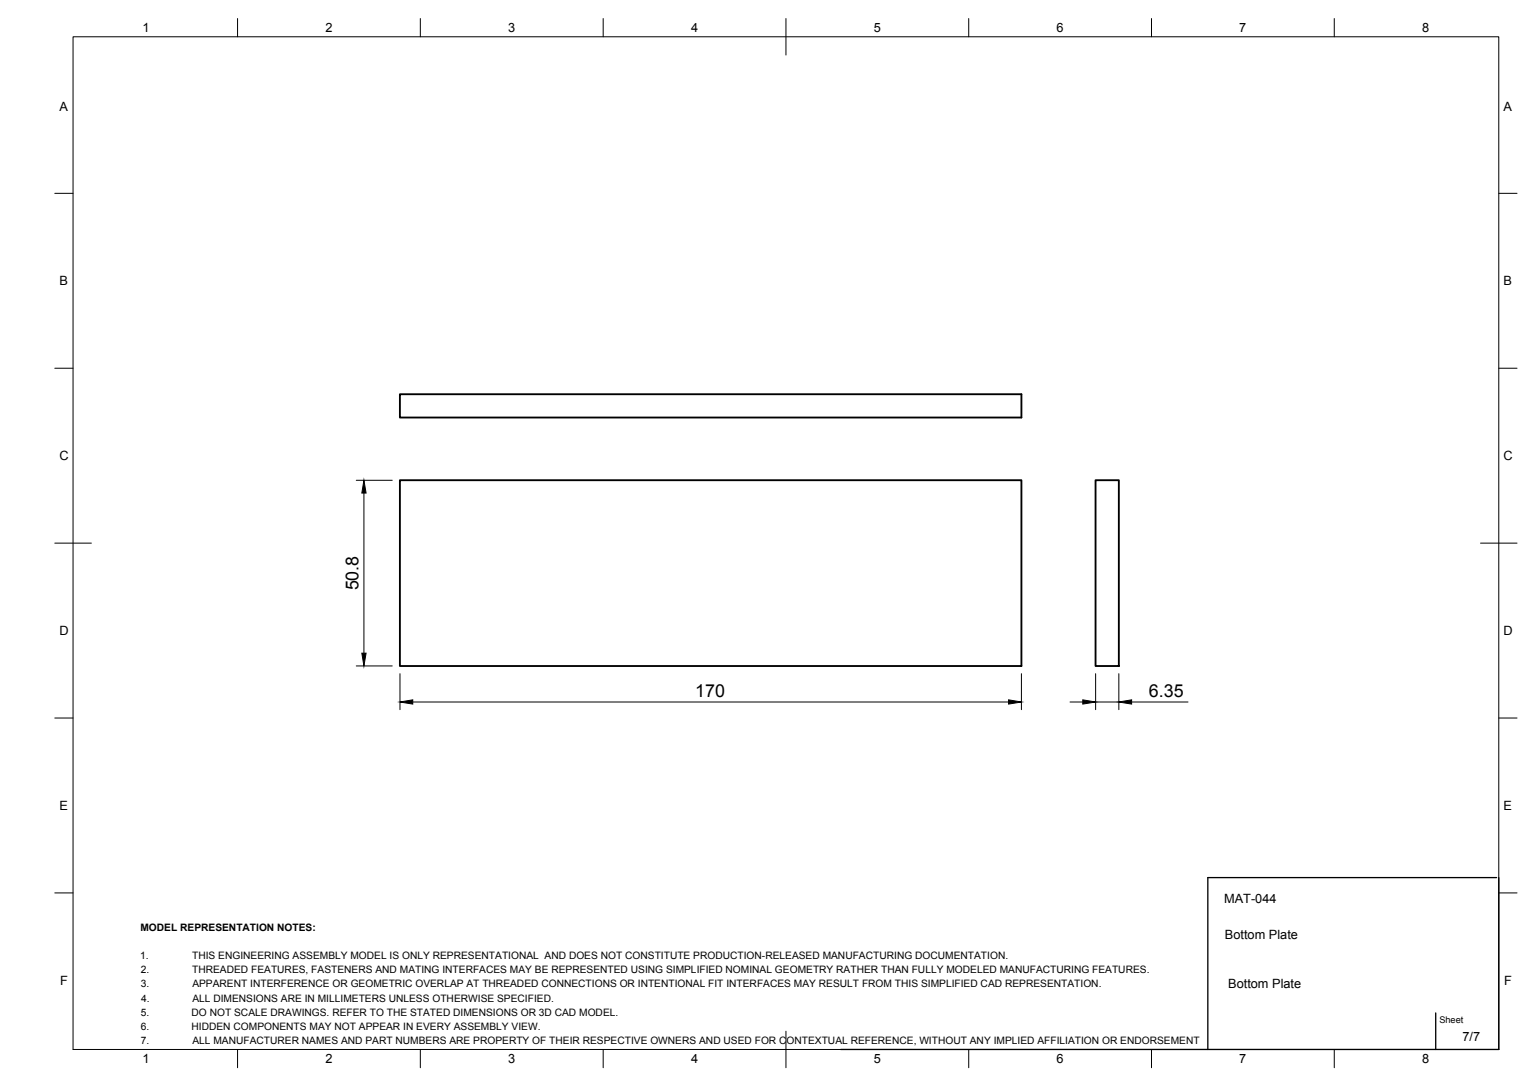
ISO-10303-21;
HEADER;
/* Generated by software containing ST-Developer
 * from STEP Tools, Inc. (www.steptools.com) 
 */

FILE_DESCRIPTION(
/* description */ ('STEP AP214'),
/* implementation_level */ '2;1');

FILE_NAME(
/* name */ 'Bottom Plate.step',
/* time_stamp */ '2026-11-14T22:20:24-08:00',
/* author */ (''),
/* organization */ (''),
/* preprocessor_version */ 'ST-DEVELOPER v20.2',
/* originating_system */ 'Autodesk Translation Framework v15.17.0.0',
/* authorisation */ '');

FILE_SCHEMA (('AUTOMOTIVE_DESIGN { 1 0 10303 214 3 1 1 }'));
ENDSEC;

DATA;
#10=MECHANICAL_DESIGN_GEOMETRIC_PRESENTATION_REPRESENTATION('',(#85),#2794);
#75=SHAPE_REPRESENTATION_RELATIONSHIP('SRR','None',#2830,#80);
#80=ADVANCED_BREP_SHAPE_REPRESENTATION('',(#90),#2792);
#85=STYLED_ITEM('',(#2863),#90);
#90=MANIFOLD_SOLID_BREP('Body1',#1644);
#178=PLANE('',#1823);
#179=PLANE('',#1824);
#180=PLANE('',#1825);
#181=PLANE('',#1826);
#182=PLANE('',#1827);
#183=PLANE('',#1828);
#266=FACE_OUTER_BOUND('',#379,.T.);
#267=FACE_OUTER_BOUND('',#380,.T.);
#268=FACE_OUTER_BOUND('',#381,.T.);
#269=FACE_OUTER_BOUND('',#382,.T.);
#270=FACE_OUTER_BOUND('',#383,.T.);
#271=FACE_OUTER_BOUND('',#384,.T.);
#379=EDGE_LOOP('',(#1490,#1491,#1492,#1493));
#380=EDGE_LOOP('',(#1494,#1495,#1496,#1497));
#381=EDGE_LOOP('',(#1498,#1499,#1500,#1501));
#382=EDGE_LOOP('',(#1502,#1503,#1504,#1505));
#383=EDGE_LOOP('',(#1506,#1507,#1508,#1509));
#384=EDGE_LOOP('',(#1510,#1511,#1512,#1513));
#546=LINE('',#2724,#715);
#547=LINE('',#2726,#716);
#548=LINE('',#2728,#717);
#549=LINE('',#2729,#718);
#550=LINE('',#2732,#719);
#551=LINE('',#2734,#720);
#552=LINE('',#2735,#721);
#553=LINE('',#2738,#722);
#554=LINE('',#2740,#723);
#555=LINE('',#2741,#724);
#556=LINE('',#2743,#725);
#557=LINE('',#2744,#726);
#715=VECTOR('',#2253,1000.);
#716=VECTOR('',#2254,1000.);
#717=VECTOR('',#2255,1000.);
#718=VECTOR('',#2256,1000.);
#719=VECTOR('',#2259,1000.);
#720=VECTOR('',#2260,1000.);
#721=VECTOR('',#2261,1000.);
#722=VECTOR('',#2264,1000.);
#723=VECTOR('',#2265,1000.);
#724=VECTOR('',#2266,1000.);
#725=VECTOR('',#2269,1000.);
#726=VECTOR('',#2270,1000.);
#887=VERTEX_POINT('',#2722);
#888=VERTEX_POINT('',#2723);
#889=VERTEX_POINT('',#2725);
#890=VERTEX_POINT('',#2727);
#891=VERTEX_POINT('',#2731);
#892=VERTEX_POINT('',#2733);
#893=VERTEX_POINT('',#2737);
#894=VERTEX_POINT('',#2739);
#1090=EDGE_CURVE('',#887,#888,#546,.T.);
#1091=EDGE_CURVE('',#889,#888,#547,.T.);
#1092=EDGE_CURVE('',#890,#889,#548,.T.);
#1093=EDGE_CURVE('',#890,#887,#549,.T.);
#1094=EDGE_CURVE('',#888,#891,#550,.T.);
#1095=EDGE_CURVE('',#892,#891,#551,.T.);
#1096=EDGE_CURVE('',#889,#892,#552,.T.);
#1097=EDGE_CURVE('',#891,#893,#553,.T.);
#1098=EDGE_CURVE('',#894,#893,#554,.T.);
#1099=EDGE_CURVE('',#892,#894,#555,.T.);
#1100=EDGE_CURVE('',#893,#887,#556,.T.);
#1101=EDGE_CURVE('',#894,#890,#557,.T.);
#1490=ORIENTED_EDGE('',*,*,#1090,.T.);
#1491=ORIENTED_EDGE('',*,*,#1091,.F.);
#1492=ORIENTED_EDGE('',*,*,#1092,.F.);
#1493=ORIENTED_EDGE('',*,*,#1093,.T.);
#1494=ORIENTED_EDGE('',*,*,#1094,.T.);
#1495=ORIENTED_EDGE('',*,*,#1095,.F.);
#1496=ORIENTED_EDGE('',*,*,#1096,.F.);
#1497=ORIENTED_EDGE('',*,*,#1091,.T.);
#1498=ORIENTED_EDGE('',*,*,#1097,.T.);
#1499=ORIENTED_EDGE('',*,*,#1098,.F.);
#1500=ORIENTED_EDGE('',*,*,#1099,.F.);
#1501=ORIENTED_EDGE('',*,*,#1095,.T.);
#1502=ORIENTED_EDGE('',*,*,#1100,.T.);
#1503=ORIENTED_EDGE('',*,*,#1093,.F.);
#1504=ORIENTED_EDGE('',*,*,#1101,.F.);
#1505=ORIENTED_EDGE('',*,*,#1098,.T.);
#1506=ORIENTED_EDGE('',*,*,#1092,.T.);
#1507=ORIENTED_EDGE('',*,*,#1096,.T.);
#1508=ORIENTED_EDGE('',*,*,#1099,.T.);
#1509=ORIENTED_EDGE('',*,*,#1101,.T.);
#1510=ORIENTED_EDGE('',*,*,#1090,.F.);
#1511=ORIENTED_EDGE('',*,*,#1100,.F.);
#1512=ORIENTED_EDGE('',*,*,#1097,.F.);
#1513=ORIENTED_EDGE('',*,*,#1094,.F.);
#1630=ADVANCED_FACE('',(#266),#178,.F.);
#1631=ADVANCED_FACE('',(#267),#179,.F.);
#1632=ADVANCED_FACE('',(#268),#180,.F.);
#1633=ADVANCED_FACE('',(#269),#181,.F.);
#1634=ADVANCED_FACE('',(#270),#182,.F.);
#1635=ADVANCED_FACE('',(#271),#183,.T.);
#1644=CLOSED_SHELL('',(#1630,#1631,#1632,#1633,#1634,#1635));
#1822=AXIS2_PLACEMENT_3D('',#2720,#2249,#2250);
#1823=AXIS2_PLACEMENT_3D('',#2721,#2251,#2252);
#1824=AXIS2_PLACEMENT_3D('',#2730,#2257,#2258);
#1825=AXIS2_PLACEMENT_3D('',#2736,#2262,#2263);
#1826=AXIS2_PLACEMENT_3D('',#2742,#2267,#2268);
#1827=AXIS2_PLACEMENT_3D('',#2745,#2271,#2272);
#1828=AXIS2_PLACEMENT_3D('',#2746,#2273,#2274);
#2249=DIRECTION('axis',(0.,0.,1.));
#2250=DIRECTION('refdir',(1.,0.,0.));
#2251=DIRECTION('center_axis',(1.,-4.72726926582308E-31,-2.33146835171283E-15));
#2252=DIRECTION('ref_axis',(-2.33146835171283E-15,3.69778549322349E-30,
-1.));
#2253=DIRECTION('',(4.7272692658233E-31,-1.,3.54987407349459E-30));
#2254=DIRECTION('',(-2.33146835171283E-15,3.69778549322349E-30,-1.));
#2255=DIRECTION('',(4.7272692658233E-31,-1.,3.54987407349459E-30));
#2256=DIRECTION('',(-2.33146835171283E-15,3.69778549322349E-30,-1.));
#2257=DIRECTION('center_axis',(-4.72726926582313E-31,1.,3.69778549322349E-30));
#2258=DIRECTION('ref_axis',(2.33146835171283E-15,-3.69778549322349E-30,
1.));
#2259=DIRECTION('',(1.,-4.72726926582326E-31,2.33146835171283E-15));
#2260=DIRECTION('',(-2.33146835171283E-15,3.69778549322349E-30,-1.));
#2261=DIRECTION('',(1.,-4.72726926582326E-31,2.33146835171283E-15));
#2262=DIRECTION('center_axis',(-1.,4.72726926582308E-31,2.33146835171283E-15));
#2263=DIRECTION('ref_axis',(2.33146835171283E-15,-3.69778549322349E-30,
1.));
#2264=DIRECTION('',(-4.7272692658233E-31,1.,-3.54987407349459E-30));
#2265=DIRECTION('',(-2.33146835171283E-15,3.69778549322349E-30,-1.));
#2266=DIRECTION('',(-4.7272692658233E-31,1.,-3.54987407349459E-30));
#2267=DIRECTION('center_axis',(4.72726926582313E-31,-1.,-3.69778549322349E-30));
#2268=DIRECTION('ref_axis',(-2.33146835171283E-15,3.69778549322349E-30,
-1.));
#2269=DIRECTION('',(-1.,4.72726926582326E-31,-2.33146835171283E-15));
#2270=DIRECTION('',(-1.,4.72726926582326E-31,-2.33146835171283E-15));
#2271=DIRECTION('center_axis',(2.33146835171283E-15,3.69778549322349E-30,
-1.));
#2272=DIRECTION('ref_axis',(-1.,4.72726926582325E-31,-2.33146835171283E-15));
#2273=DIRECTION('center_axis',(2.33146835171283E-15,3.69778549322349E-30,
-1.));
#2274=DIRECTION('ref_axis',(-1.,4.72726926582325E-31,-2.33146835171283E-15));
#2720=CARTESIAN_POINT('',(0.,0.,0.));
#2721=CARTESIAN_POINT('Origin',(0.,0.,6.35));
#2722=CARTESIAN_POINT('',(0.,50.7999999999971,-3.19189119579733E-13));
#2723=CARTESIAN_POINT('',(0.,0.,0.));
#2724=CARTESIAN_POINT('',(0.,0.,0.));
#2725=CARTESIAN_POINT('',(0.,0.,6.35));
#2726=CARTESIAN_POINT('',(0.,0.,6.35));
#2727=CARTESIAN_POINT('',(0.,50.7999999999971,6.35000000000001));
#2728=CARTESIAN_POINT('',(0.,0.,6.35));
#2729=CARTESIAN_POINT('',(0.,50.7999999999971,6.35000000000001));
#2730=CARTESIAN_POINT('Origin',(0.,0.,6.35));
#2731=CARTESIAN_POINT('',(170.,0.,5.20417042793042E-13));
#2732=CARTESIAN_POINT('',(0.,0.,0.));
#2733=CARTESIAN_POINT('',(170.,0.,6.35000000000051));
#2734=CARTESIAN_POINT('',(170.,0.,6.35000000000051));
#2735=CARTESIAN_POINT('',(0.,0.,6.35));
#2736=CARTESIAN_POINT('Origin',(170.,0.,6.35000000000051));
#2737=CARTESIAN_POINT('',(170.,50.7999999999971,4.92661467177413E-13));
#2738=CARTESIAN_POINT('',(170.,0.,5.20417042793042E-13));
#2739=CARTESIAN_POINT('',(170.,50.7999999999971,6.3500000000005));
#2740=CARTESIAN_POINT('',(170.,50.7999999999971,6.3500000000005));
#2741=CARTESIAN_POINT('',(170.,0.,6.35000000000051));
#2742=CARTESIAN_POINT('Origin',(0.,50.7999999999971,6.35000000000001));
#2743=CARTESIAN_POINT('',(0.,50.7999999999971,-3.19189119579733E-13));
#2744=CARTESIAN_POINT('',(0.,50.7999999999971,6.35000000000001));
#2745=CARTESIAN_POINT('Origin',(0.,0.,6.35));
#2746=CARTESIAN_POINT('Origin',(0.,0.,0.));
#2785=UNCERTAINTY_MEASURE_WITH_UNIT(LENGTH_MEASURE(0.01),#2795,
'DISTANCE_ACCURACY_VALUE',
'Maximum model space distance between geometric entities at asserted c
onnectivities');
#2787=UNCERTAINTY_MEASURE_WITH_UNIT(LENGTH_MEASURE(0.01),#2795,
'DISTANCE_ACCURACY_VALUE',
'Maximum model space distance between geometric entities at asserted c
onnectivities');
#2792=(
GEOMETRIC_REPRESENTATION_CONTEXT(3)
GLOBAL_UNCERTAINTY_ASSIGNED_CONTEXT((#2785))
GLOBAL_UNIT_ASSIGNED_CONTEXT((#2795,#2797,#2798))
REPRESENTATION_CONTEXT('','3D')
);
#2794=(
GEOMETRIC_REPRESENTATION_CONTEXT(3)
GLOBAL_UNCERTAINTY_ASSIGNED_CONTEXT((#2787))
GLOBAL_UNIT_ASSIGNED_CONTEXT((#2795,#2797,#2798))
REPRESENTATION_CONTEXT('','3D')
);
#2795=(
LENGTH_UNIT()
NAMED_UNIT(*)
SI_UNIT(.MILLI.,.METRE.)
);
#2797=(
NAMED_UNIT(*)
PLANE_ANGLE_UNIT()
SI_UNIT($,.RADIAN.)
);
#2798=(
NAMED_UNIT(*)
SI_UNIT($,.STERADIAN.)
SOLID_ANGLE_UNIT()
);
#2803=SHAPE_DEFINITION_REPRESENTATION(#2809,#2830);
#2809=PRODUCT_DEFINITION_SHAPE('',$,#2837);
#2830=SHAPE_REPRESENTATION('',(#1822),#2792);
#2832=PRODUCT_DEFINITION_CONTEXT('part definition',#2852,'design');
#2837=PRODUCT_DEFINITION('Bottom Plate','Bottom Plate',#2843,#2832);
#2843=PRODUCT_DEFINITION_FORMATION('',$,#2858);
#2852=APPLICATION_CONTEXT(
'Core Data for Automotive Mechanical Design Process');
#2853=PRODUCT_CONTEXT('part definition',#2852,'mechanical');
#2858=PRODUCT('Bottom Plate','Bottom Plate',$,(#2853));
#2863=PRESENTATION_STYLE_ASSIGNMENT((#2867));
#2867=SURFACE_STYLE_USAGE(.BOTH.,#2871);
#2871=SURFACE_SIDE_STYLE('',(#2875));
#2875=SURFACE_STYLE_FILL_AREA(#2879);
#2879=FILL_AREA_STYLE('Opaque(227,224,212)',(#2883));
#2883=FILL_AREA_STYLE_COLOUR('Opaque(227,224,212)',#2887);
#2887=COLOUR_RGB('Opaque(227,224,212)',0.890196078431372,0.87843137254902,
0.831372549019608);
ENDSEC;
END-ISO-10303-21;
